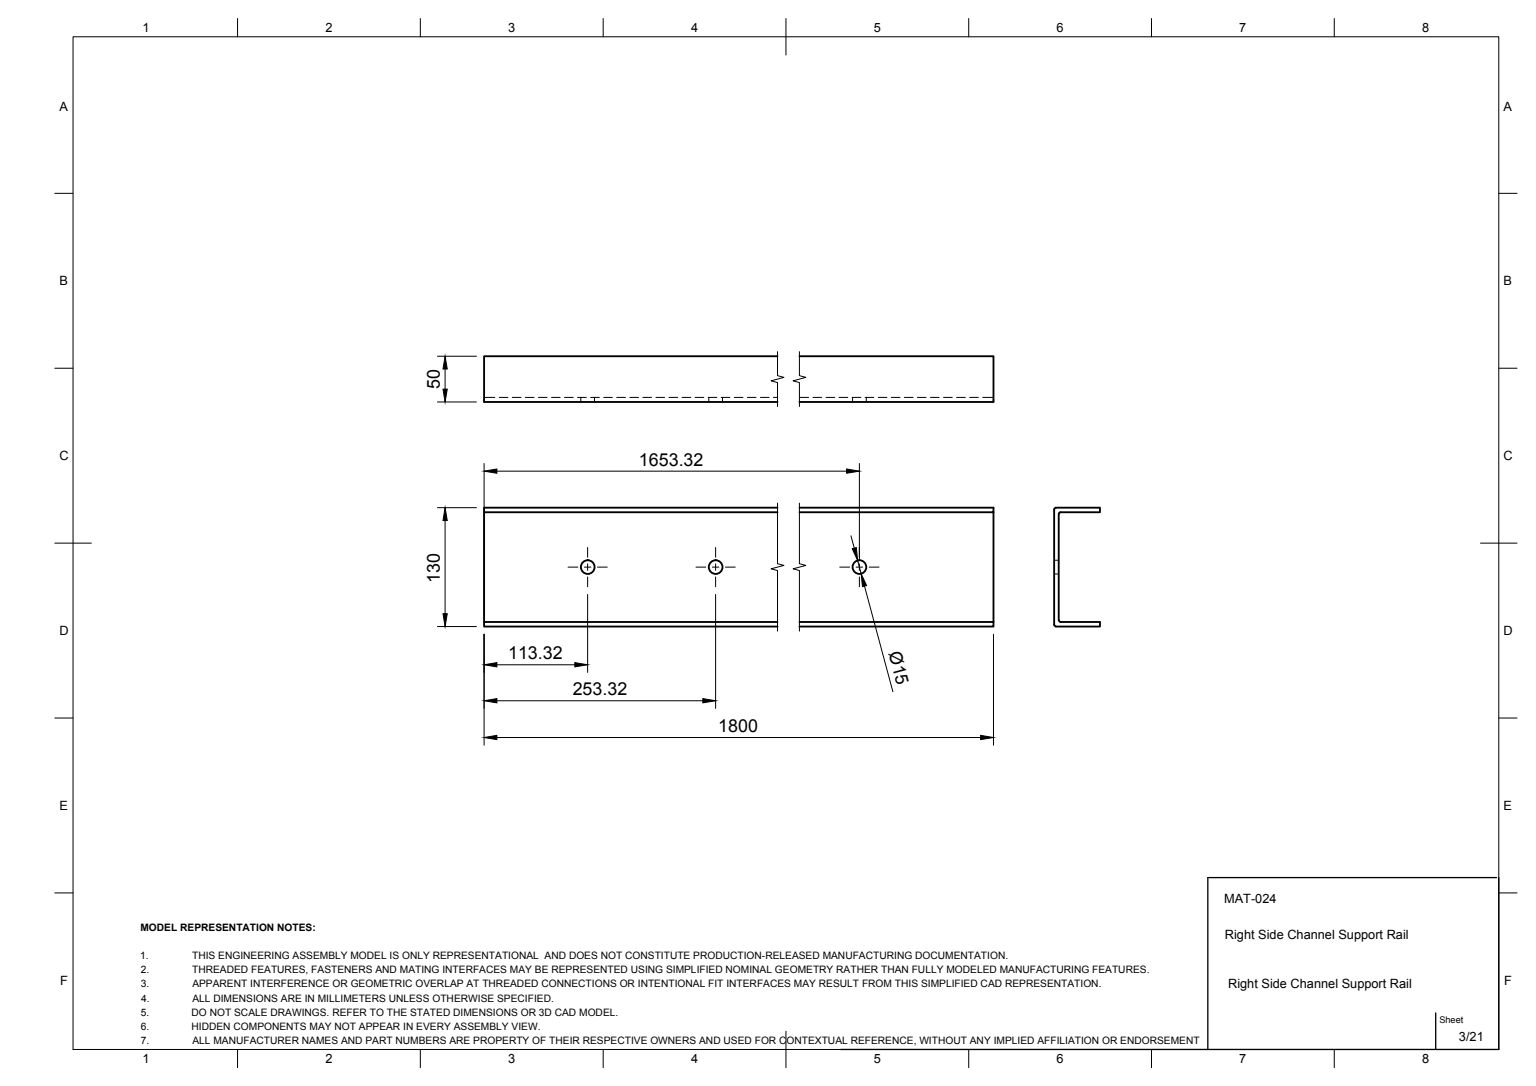
ISO-10303-21;
HEADER;
/* Generated by software containing ST-Developer
 * from STEP Tools, Inc. (www.steptools.com) 
 */

FILE_DESCRIPTION(
/* description */ ('STEP AP214'),
/* implementation_level */ '2;1');

FILE_NAME(
/* name */ 'Right Side Channel Support Rail.step',
/* time_stamp */ '2026-11-14T06:34:07-08:00',
/* author */ (''),
/* organization */ (''),
/* preprocessor_version */ 'ST-DEVELOPER v20.2',
/* originating_system */ 'Autodesk Translation Framework v15.17.0.0',
/* authorisation */ '');

FILE_SCHEMA (('AUTOMOTIVE_DESIGN { 1 0 10303 214 3 1 1 }'));
ENDSEC;

DATA;
#10=MECHANICAL_DESIGN_GEOMETRIC_PRESENTATION_REPRESENTATION('',(#7256),#310623);
#7222=SHAPE_REPRESENTATION_RELATIONSHIP('SRR','None',#310894,#7239);
#7239=ADVANCED_BREP_SHAPE_REPRESENTATION('',(#7324),#310603);
#7256=STYLED_ITEM('',(#311003),#7324);
#7324=MANIFOLD_SOLID_BREP('Body1',#93706);
#7391=FACE_BOUND('',#14442,.T.);
#7392=FACE_BOUND('',#14443,.T.);
#7393=FACE_BOUND('',#14444,.T.);
#7394=FACE_BOUND('',#14445,.T.);
#7395=FACE_BOUND('',#14446,.T.);
#7396=FACE_BOUND('',#14447,.T.);
#7397=FACE_BOUND('',#14448,.T.);
#7398=FACE_BOUND('',#14449,.T.);
#7399=FACE_BOUND('',#14450,.T.);
#7400=FACE_BOUND('',#14451,.T.);
#7401=FACE_BOUND('',#14452,.T.);
#7402=FACE_BOUND('',#14453,.T.);
#7403=FACE_BOUND('',#14458,.T.);
#7404=FACE_BOUND('',#14459,.T.);
#7405=FACE_BOUND('',#14460,.T.);
#7406=FACE_BOUND('',#14461,.T.);
#7407=FACE_BOUND('',#14462,.T.);
#7408=FACE_BOUND('',#14463,.T.);
#7409=FACE_BOUND('',#14464,.T.);
#7410=FACE_BOUND('',#14465,.T.);
#7411=FACE_BOUND('',#14466,.T.);
#7412=FACE_BOUND('',#14467,.T.);
#7413=FACE_BOUND('',#14468,.T.);
#7414=FACE_BOUND('',#14469,.T.);
#7706=PLANE('',#94001);
#7707=PLANE('',#94002);
#7708=PLANE('',#94003);
#7709=PLANE('',#94004);
#7710=PLANE('',#94005);
#7711=PLANE('',#94006);
#7712=PLANE('',#94007);
#7713=PLANE('',#94008);
#7714=PLANE('',#94009);
#7715=PLANE('',#94014);
#8688=FACE_OUTER_BOUND('',#14427,.T.);
#8689=FACE_OUTER_BOUND('',#14428,.T.);
#8690=FACE_OUTER_BOUND('',#14429,.T.);
#8691=FACE_OUTER_BOUND('',#14430,.T.);
#8692=FACE_OUTER_BOUND('',#14431,.T.);
#8693=FACE_OUTER_BOUND('',#14432,.T.);
#8694=FACE_OUTER_BOUND('',#14433,.T.);
#8695=FACE_OUTER_BOUND('',#14434,.T.);
#8696=FACE_OUTER_BOUND('',#14435,.T.);
#8697=FACE_OUTER_BOUND('',#14436,.T.);
#8698=FACE_OUTER_BOUND('',#14437,.T.);
#8699=FACE_OUTER_BOUND('',#14438,.T.);
#8700=FACE_OUTER_BOUND('',#14439,.T.);
#8701=FACE_OUTER_BOUND('',#14440,.T.);
#8702=FACE_OUTER_BOUND('',#14441,.T.);
#8703=FACE_OUTER_BOUND('',#14454,.T.);
#8704=FACE_OUTER_BOUND('',#14455,.T.);
#8705=FACE_OUTER_BOUND('',#14456,.T.);
#8706=FACE_OUTER_BOUND('',#14457,.T.);
#8707=FACE_OUTER_BOUND('',#14470,.T.);
#8708=FACE_OUTER_BOUND('',#14471,.T.);
#8709=FACE_OUTER_BOUND('',#14472,.T.);
#8710=FACE_OUTER_BOUND('',#14473,.T.);
#8711=FACE_OUTER_BOUND('',#14474,.T.);
#8712=FACE_OUTER_BOUND('',#14475,.T.);
#8713=FACE_OUTER_BOUND('',#14476,.T.);
#14427=EDGE_LOOP('',(#57657,#57658,#57659,#57660));
#14428=EDGE_LOOP('',(#57661,#57662,#57663,#57664));
#14429=EDGE_LOOP('',(#57665,#57666,#57667,#57668));
#14430=EDGE_LOOP('',(#57669,#57670,#57671,#57672));
#14431=EDGE_LOOP('',(#57673,#57674,#57675,#57676));
#14432=EDGE_LOOP('',(#57677,#57678,#57679,#57680));
#14433=EDGE_LOOP('',(#57681,#57682,#57683,#57684));
#14434=EDGE_LOOP('',(#57685,#57686,#57687,#57688));
#14435=EDGE_LOOP('',(#57689,#57690,#57691,#57692));
#14436=EDGE_LOOP('',(#57693,#57694,#57695,#57696));
#14437=EDGE_LOOP('',(#57697,#57698,#57699,#57700));
#14438=EDGE_LOOP('',(#57701,#57702,#57703,#57704));
#14439=EDGE_LOOP('',(#57705,#57706,#57707,#57708));
#14440=EDGE_LOOP('',(#57709,#57710,#57711,#57712));
#14441=EDGE_LOOP('',(#57713,#57714,#57715,#57716));
#14442=EDGE_LOOP('',(#57717));
#14443=EDGE_LOOP('',(#57718));
#14444=EDGE_LOOP('',(#57719));
#14445=EDGE_LOOP('',(#57720));
#14446=EDGE_LOOP('',(#57721));
#14447=EDGE_LOOP('',(#57722));
#14448=EDGE_LOOP('',(#57723));
#14449=EDGE_LOOP('',(#57724));
#14450=EDGE_LOOP('',(#57725));
#14451=EDGE_LOOP('',(#57726));
#14452=EDGE_LOOP('',(#57727));
#14453=EDGE_LOOP('',(#57728));
#14454=EDGE_LOOP('',(#57729,#57730,#57731,#57732));
#14455=EDGE_LOOP('',(#57733,#57734,#57735,#57736));
#14456=EDGE_LOOP('',(#57737,#57738,#57739,#57740));
#14457=EDGE_LOOP('',(#57741,#57742,#57743,#57744));
#14458=EDGE_LOOP('',(#57745));
#14459=EDGE_LOOP('',(#57746));
#14460=EDGE_LOOP('',(#57747));
#14461=EDGE_LOOP('',(#57748));
#14462=EDGE_LOOP('',(#57749));
#14463=EDGE_LOOP('',(#57750));
#14464=EDGE_LOOP('',(#57751));
#14465=EDGE_LOOP('',(#57752));
#14466=EDGE_LOOP('',(#57753));
#14467=EDGE_LOOP('',(#57754));
#14468=EDGE_LOOP('',(#57755));
#14469=EDGE_LOOP('',(#57756));
#14470=EDGE_LOOP('',(#57757,#57758,#57759,#57760));
#14471=EDGE_LOOP('',(#57761,#57762,#57763,#57764,#57765,#57766,#57767,#57768,
#57769,#57770,#57771,#57772));
#14472=EDGE_LOOP('',(#57773,#57774,#57775,#57776,#57777,#57778,#57779,#57780,
#57781,#57782,#57783,#57784));
#14473=EDGE_LOOP('',(#57785,#57786,#57787,#57788));
#14474=EDGE_LOOP('',(#57789,#57790,#57791,#57792));
#14475=EDGE_LOOP('',(#57793,#57794,#57795,#57796));
#14476=EDGE_LOOP('',(#57797,#57798,#57799,#57800));
#20481=LINE('',#131019,#24828);
#20482=LINE('',#131025,#24829);
#20483=LINE('',#131031,#24830);
#20484=LINE('',#131037,#24831);
#20485=LINE('',#131043,#24832);
#20486=LINE('',#131049,#24833);
#20487=LINE('',#131055,#24834);
#20488=LINE('',#131061,#24835);
#20489=LINE('',#131067,#24836);
#20490=LINE('',#131073,#24837);
#20491=LINE('',#131079,#24838);
#20492=LINE('',#131085,#24839);
#20493=LINE('',#131090,#24840);
#20494=LINE('',#131092,#24841);
#20495=LINE('',#131094,#24842);
#20496=LINE('',#131095,#24843);
#20497=LINE('',#131098,#24844);
#20498=LINE('',#131100,#24845);
#20499=LINE('',#131101,#24846);
#20500=LINE('',#131105,#24847);
#20501=LINE('',#131107,#24848);
#20502=LINE('',#131109,#24849);
#20503=LINE('',#131110,#24850);
#20504=LINE('',#131114,#24851);
#20505=LINE('',#131116,#24852);
#20506=LINE('',#131118,#24853);
#20507=LINE('',#131119,#24854);
#20508=LINE('',#131122,#24855);
#20509=LINE('',#131124,#24856);
#20510=LINE('',#131125,#24857);
#20511=LINE('',#131128,#24858);
#20512=LINE('',#131130,#24859);
#20513=LINE('',#131131,#24860);
#20514=LINE('',#131135,#24861);
#20515=LINE('',#131137,#24862);
#20516=LINE('',#131139,#24863);
#20517=LINE('',#131140,#24864);
#20518=LINE('',#131143,#24865);
#20519=LINE('',#131145,#24866);
#20520=LINE('',#131146,#24867);
#24828=VECTOR('',#104872,7.5);
#24829=VECTOR('',#104879,7.5);
#24830=VECTOR('',#104886,7.50000000000001);
#24831=VECTOR('',#104893,7.5);
#24832=VECTOR('',#104900,7.50000000000001);
#24833=VECTOR('',#104907,7.5);
#24834=VECTOR('',#104914,7.5);
#24835=VECTOR('',#104921,7.5);
#24836=VECTOR('',#104928,7.5);
#24837=VECTOR('',#104935,7.5);
#24838=VECTOR('',#104942,7.5);
#24839=VECTOR('',#104949,7.50000000000001);
#24840=VECTOR('',#104954,1000.);
#24841=VECTOR('',#104955,1000.);
#24842=VECTOR('',#104956,1000.);
#24843=VECTOR('',#104957,1000.);
#24844=VECTOR('',#104960,1000.);
#24845=VECTOR('',#104961,1000.);
#24846=VECTOR('',#104962,1000.);
#24847=VECTOR('',#104965,1000.);
#24848=VECTOR('',#104966,1000.);
#24849=VECTOR('',#104967,1000.);
#24850=VECTOR('',#104968,1000.);
#24851=VECTOR('',#104971,1000.);
#24852=VECTOR('',#104972,1000.);
#24853=VECTOR('',#104973,1000.);
#24854=VECTOR('',#104974,1000.);
#24855=VECTOR('',#104977,1000.);
#24856=VECTOR('',#104978,1000.);
#24857=VECTOR('',#104979,1000.);
#24858=VECTOR('',#104982,1000.);
#24859=VECTOR('',#104983,1000.);
#24860=VECTOR('',#104984,1000.);
#24861=VECTOR('',#104987,1000.);
#24862=VECTOR('',#104988,1000.);
#24863=VECTOR('',#104989,1000.);
#24864=VECTOR('',#104990,1000.);
#24865=VECTOR('',#104993,1000.);
#24866=VECTOR('',#104994,1000.);
#24867=VECTOR('',#104995,1000.);
#29175=CIRCLE('',#93966,7.5);
#29176=CIRCLE('',#93967,7.5);
#29177=CIRCLE('',#93969,7.5);
#29178=CIRCLE('',#93970,7.5);
#29179=CIRCLE('',#93972,7.50000000000001);
#29180=CIRCLE('',#93973,7.50000000000001);
#29181=CIRCLE('',#93975,7.5);
#29182=CIRCLE('',#93976,7.5);
#29183=CIRCLE('',#93978,7.50000000000001);
#29184=CIRCLE('',#93979,7.50000000000001);
#29185=CIRCLE('',#93981,7.5);
#29186=CIRCLE('',#93982,7.5);
#29187=CIRCLE('',#93984,7.5);
#29188=CIRCLE('',#93985,7.5);
#29189=CIRCLE('',#93987,7.5);
#29190=CIRCLE('',#93988,7.5);
#29191=CIRCLE('',#93990,7.5);
#29192=CIRCLE('',#93991,7.5);
#29193=CIRCLE('',#93993,7.5);
#29194=CIRCLE('',#93994,7.5);
#29195=CIRCLE('',#93996,7.5);
#29196=CIRCLE('',#93997,7.5);
#29197=CIRCLE('',#93999,7.50000000000001);
#29198=CIRCLE('',#94000,7.50000000000001);
#29199=CIRCLE('',#94010,2.);
#29200=CIRCLE('',#94011,2.);
#29201=CIRCLE('',#94012,2.);
#29202=CIRCLE('',#94013,2.);
#29203=CIRCLE('',#94015,2.);
#29204=CIRCLE('',#94016,2.);
#29205=CIRCLE('',#94017,2.);
#29206=CIRCLE('',#94018,2.);
#35105=VERTEX_POINT('',#131016);
#35106=VERTEX_POINT('',#131018);
#35107=VERTEX_POINT('',#131022);
#35108=VERTEX_POINT('',#131024);
#35109=VERTEX_POINT('',#131028);
#35110=VERTEX_POINT('',#131030);
#35111=VERTEX_POINT('',#131034);
#35112=VERTEX_POINT('',#131036);
#35113=VERTEX_POINT('',#131040);
#35114=VERTEX_POINT('',#131042);
#35115=VERTEX_POINT('',#131046);
#35116=VERTEX_POINT('',#131048);
#35117=VERTEX_POINT('',#131052);
#35118=VERTEX_POINT('',#131054);
#35119=VERTEX_POINT('',#131058);
#35120=VERTEX_POINT('',#131060);
#35121=VERTEX_POINT('',#131064);
#35122=VERTEX_POINT('',#131066);
#35123=VERTEX_POINT('',#131070);
#35124=VERTEX_POINT('',#131072);
#35125=VERTEX_POINT('',#131076);
#35126=VERTEX_POINT('',#131078);
#35127=VERTEX_POINT('',#131082);
#35128=VERTEX_POINT('',#131084);
#35129=VERTEX_POINT('',#131088);
#35130=VERTEX_POINT('',#131089);
#35131=VERTEX_POINT('',#131091);
#35132=VERTEX_POINT('',#131093);
#35133=VERTEX_POINT('',#131097);
#35134=VERTEX_POINT('',#131099);
#35135=VERTEX_POINT('',#131103);
#35136=VERTEX_POINT('',#131104);
#35137=VERTEX_POINT('',#131106);
#35138=VERTEX_POINT('',#131108);
#35139=VERTEX_POINT('',#131112);
#35140=VERTEX_POINT('',#131113);
#35141=VERTEX_POINT('',#131115);
#35142=VERTEX_POINT('',#131117);
#35143=VERTEX_POINT('',#131121);
#35144=VERTEX_POINT('',#131123);
#35145=VERTEX_POINT('',#131127);
#35146=VERTEX_POINT('',#131129);
#35147=VERTEX_POINT('',#131133);
#35148=VERTEX_POINT('',#131134);
#35149=VERTEX_POINT('',#131136);
#35150=VERTEX_POINT('',#131138);
#35151=VERTEX_POINT('',#131142);
#35152=VERTEX_POINT('',#131144);
#43608=EDGE_CURVE('',#35105,#35105,#29175,.T.);
#43609=EDGE_CURVE('',#35105,#35106,#20481,.T.);
#43610=EDGE_CURVE('',#35106,#35106,#29176,.T.);
#43611=EDGE_CURVE('',#35107,#35107,#29177,.T.);
#43612=EDGE_CURVE('',#35107,#35108,#20482,.T.);
#43613=EDGE_CURVE('',#35108,#35108,#29178,.T.);
#43614=EDGE_CURVE('',#35109,#35109,#29179,.T.);
#43615=EDGE_CURVE('',#35109,#35110,#20483,.T.);
#43616=EDGE_CURVE('',#35110,#35110,#29180,.T.);
#43617=EDGE_CURVE('',#35111,#35111,#29181,.T.);
#43618=EDGE_CURVE('',#35111,#35112,#20484,.T.);
#43619=EDGE_CURVE('',#35112,#35112,#29182,.T.);
#43620=EDGE_CURVE('',#35113,#35113,#29183,.T.);
#43621=EDGE_CURVE('',#35113,#35114,#20485,.T.);
#43622=EDGE_CURVE('',#35114,#35114,#29184,.T.);
#43623=EDGE_CURVE('',#35115,#35115,#29185,.T.);
#43624=EDGE_CURVE('',#35115,#35116,#20486,.T.);
#43625=EDGE_CURVE('',#35116,#35116,#29186,.T.);
#43626=EDGE_CURVE('',#35117,#35117,#29187,.T.);
#43627=EDGE_CURVE('',#35117,#35118,#20487,.T.);
#43628=EDGE_CURVE('',#35118,#35118,#29188,.T.);
#43629=EDGE_CURVE('',#35119,#35119,#29189,.T.);
#43630=EDGE_CURVE('',#35119,#35120,#20488,.T.);
#43631=EDGE_CURVE('',#35120,#35120,#29190,.T.);
#43632=EDGE_CURVE('',#35121,#35121,#29191,.T.);
#43633=EDGE_CURVE('',#35121,#35122,#20489,.T.);
#43634=EDGE_CURVE('',#35122,#35122,#29192,.T.);
#43635=EDGE_CURVE('',#35123,#35123,#29193,.T.);
#43636=EDGE_CURVE('',#35123,#35124,#20490,.T.);
#43637=EDGE_CURVE('',#35124,#35124,#29194,.T.);
#43638=EDGE_CURVE('',#35125,#35125,#29195,.T.);
#43639=EDGE_CURVE('',#35125,#35126,#20491,.T.);
#43640=EDGE_CURVE('',#35126,#35126,#29196,.T.);
#43641=EDGE_CURVE('',#35127,#35127,#29197,.T.);
#43642=EDGE_CURVE('',#35127,#35128,#20492,.T.);
#43643=EDGE_CURVE('',#35128,#35128,#29198,.T.);
#43644=EDGE_CURVE('',#35129,#35130,#20493,.T.);
#43645=EDGE_CURVE('',#35131,#35130,#20494,.T.);
#43646=EDGE_CURVE('',#35132,#35131,#20495,.T.);
#43647=EDGE_CURVE('',#35132,#35129,#20496,.T.);
#43648=EDGE_CURVE('',#35130,#35133,#20497,.T.);
#43649=EDGE_CURVE('',#35133,#35134,#20498,.T.);
#43650=EDGE_CURVE('',#35131,#35134,#20499,.T.);
#43651=EDGE_CURVE('',#35135,#35136,#20500,.T.);
#43652=EDGE_CURVE('',#35136,#35137,#20501,.T.);
#43653=EDGE_CURVE('',#35138,#35137,#20502,.T.);
#43654=EDGE_CURVE('',#35138,#35135,#20503,.T.);
#43655=EDGE_CURVE('',#35139,#35140,#20504,.T.);
#43656=EDGE_CURVE('',#35139,#35141,#20505,.T.);
#43657=EDGE_CURVE('',#35141,#35142,#20506,.T.);
#43658=EDGE_CURVE('',#35140,#35142,#20507,.T.);
#43659=EDGE_CURVE('',#35142,#35143,#20508,.T.);
#43660=EDGE_CURVE('',#35144,#35143,#20509,.T.);
#43661=EDGE_CURVE('',#35140,#35144,#20510,.T.);
#43662=EDGE_CURVE('',#35143,#35145,#20511,.T.);
#43663=EDGE_CURVE('',#35145,#35146,#20512,.T.);
#43664=EDGE_CURVE('',#35144,#35146,#20513,.T.);
#43665=EDGE_CURVE('',#35147,#35148,#20514,.T.);
#43666=EDGE_CURVE('',#35148,#35149,#20515,.T.);
#43667=EDGE_CURVE('',#35150,#35149,#20516,.T.);
#43668=EDGE_CURVE('',#35150,#35147,#20517,.T.);
#43669=EDGE_CURVE('',#35151,#35132,#20518,.T.);
#43670=EDGE_CURVE('',#35151,#35152,#20519,.T.);
#43671=EDGE_CURVE('',#35152,#35129,#20520,.T.);
#43672=EDGE_CURVE('',#35137,#35139,#29199,.T.);
#43673=EDGE_CURVE('',#35146,#35150,#29200,.T.);
#43674=EDGE_CURVE('',#35149,#35151,#29201,.T.);
#43675=EDGE_CURVE('',#35134,#35138,#29202,.T.);
#43676=EDGE_CURVE('',#35141,#35136,#29203,.T.);
#43677=EDGE_CURVE('',#35135,#35133,#29204,.T.);
#43678=EDGE_CURVE('',#35152,#35148,#29205,.T.);
#43679=EDGE_CURVE('',#35147,#35145,#29206,.T.);
#57657=ORIENTED_EDGE('',*,*,#43608,.F.);
#57658=ORIENTED_EDGE('',*,*,#43609,.T.);
#57659=ORIENTED_EDGE('',*,*,#43610,.T.);
#57660=ORIENTED_EDGE('',*,*,#43609,.F.);
#57661=ORIENTED_EDGE('',*,*,#43611,.F.);
#57662=ORIENTED_EDGE('',*,*,#43612,.T.);
#57663=ORIENTED_EDGE('',*,*,#43613,.T.);
#57664=ORIENTED_EDGE('',*,*,#43612,.F.);
#57665=ORIENTED_EDGE('',*,*,#43614,.F.);
#57666=ORIENTED_EDGE('',*,*,#43615,.T.);
#57667=ORIENTED_EDGE('',*,*,#43616,.T.);
#57668=ORIENTED_EDGE('',*,*,#43615,.F.);
#57669=ORIENTED_EDGE('',*,*,#43617,.F.);
#57670=ORIENTED_EDGE('',*,*,#43618,.T.);
#57671=ORIENTED_EDGE('',*,*,#43619,.T.);
#57672=ORIENTED_EDGE('',*,*,#43618,.F.);
#57673=ORIENTED_EDGE('',*,*,#43620,.F.);
#57674=ORIENTED_EDGE('',*,*,#43621,.T.);
#57675=ORIENTED_EDGE('',*,*,#43622,.T.);
#57676=ORIENTED_EDGE('',*,*,#43621,.F.);
#57677=ORIENTED_EDGE('',*,*,#43623,.F.);
#57678=ORIENTED_EDGE('',*,*,#43624,.T.);
#57679=ORIENTED_EDGE('',*,*,#43625,.T.);
#57680=ORIENTED_EDGE('',*,*,#43624,.F.);
#57681=ORIENTED_EDGE('',*,*,#43626,.F.);
#57682=ORIENTED_EDGE('',*,*,#43627,.T.);
#57683=ORIENTED_EDGE('',*,*,#43628,.T.);
#57684=ORIENTED_EDGE('',*,*,#43627,.F.);
#57685=ORIENTED_EDGE('',*,*,#43629,.F.);
#57686=ORIENTED_EDGE('',*,*,#43630,.T.);
#57687=ORIENTED_EDGE('',*,*,#43631,.T.);
#57688=ORIENTED_EDGE('',*,*,#43630,.F.);
#57689=ORIENTED_EDGE('',*,*,#43632,.F.);
#57690=ORIENTED_EDGE('',*,*,#43633,.T.);
#57691=ORIENTED_EDGE('',*,*,#43634,.T.);
#57692=ORIENTED_EDGE('',*,*,#43633,.F.);
#57693=ORIENTED_EDGE('',*,*,#43635,.F.);
#57694=ORIENTED_EDGE('',*,*,#43636,.T.);
#57695=ORIENTED_EDGE('',*,*,#43637,.T.);
#57696=ORIENTED_EDGE('',*,*,#43636,.F.);
#57697=ORIENTED_EDGE('',*,*,#43638,.F.);
#57698=ORIENTED_EDGE('',*,*,#43639,.T.);
#57699=ORIENTED_EDGE('',*,*,#43640,.T.);
#57700=ORIENTED_EDGE('',*,*,#43639,.F.);
#57701=ORIENTED_EDGE('',*,*,#43641,.F.);
#57702=ORIENTED_EDGE('',*,*,#43642,.T.);
#57703=ORIENTED_EDGE('',*,*,#43643,.T.);
#57704=ORIENTED_EDGE('',*,*,#43642,.F.);
#57705=ORIENTED_EDGE('',*,*,#43644,.T.);
#57706=ORIENTED_EDGE('',*,*,#43645,.F.);
#57707=ORIENTED_EDGE('',*,*,#43646,.F.);
#57708=ORIENTED_EDGE('',*,*,#43647,.T.);
#57709=ORIENTED_EDGE('',*,*,#43648,.T.);
#57710=ORIENTED_EDGE('',*,*,#43649,.T.);
#57711=ORIENTED_EDGE('',*,*,#43650,.F.);
#57712=ORIENTED_EDGE('',*,*,#43645,.T.);
#57713=ORIENTED_EDGE('',*,*,#43651,.T.);
#57714=ORIENTED_EDGE('',*,*,#43652,.T.);
#57715=ORIENTED_EDGE('',*,*,#43653,.F.);
#57716=ORIENTED_EDGE('',*,*,#43654,.T.);
#57717=ORIENTED_EDGE('',*,*,#43608,.T.);
#57718=ORIENTED_EDGE('',*,*,#43611,.T.);
#57719=ORIENTED_EDGE('',*,*,#43614,.T.);
#57720=ORIENTED_EDGE('',*,*,#43617,.T.);
#57721=ORIENTED_EDGE('',*,*,#43620,.T.);
#57722=ORIENTED_EDGE('',*,*,#43623,.T.);
#57723=ORIENTED_EDGE('',*,*,#43626,.T.);
#57724=ORIENTED_EDGE('',*,*,#43629,.T.);
#57725=ORIENTED_EDGE('',*,*,#43632,.T.);
#57726=ORIENTED_EDGE('',*,*,#43635,.T.);
#57727=ORIENTED_EDGE('',*,*,#43638,.T.);
#57728=ORIENTED_EDGE('',*,*,#43641,.T.);
#57729=ORIENTED_EDGE('',*,*,#43655,.F.);
#57730=ORIENTED_EDGE('',*,*,#43656,.T.);
#57731=ORIENTED_EDGE('',*,*,#43657,.T.);
#57732=ORIENTED_EDGE('',*,*,#43658,.F.);
#57733=ORIENTED_EDGE('',*,*,#43659,.T.);
#57734=ORIENTED_EDGE('',*,*,#43660,.F.);
#57735=ORIENTED_EDGE('',*,*,#43661,.F.);
#57736=ORIENTED_EDGE('',*,*,#43658,.T.);
#57737=ORIENTED_EDGE('',*,*,#43662,.T.);
#57738=ORIENTED_EDGE('',*,*,#43663,.T.);
#57739=ORIENTED_EDGE('',*,*,#43664,.F.);
#57740=ORIENTED_EDGE('',*,*,#43660,.T.);
#57741=ORIENTED_EDGE('',*,*,#43665,.T.);
#57742=ORIENTED_EDGE('',*,*,#43666,.T.);
#57743=ORIENTED_EDGE('',*,*,#43667,.F.);
#57744=ORIENTED_EDGE('',*,*,#43668,.T.);
#57745=ORIENTED_EDGE('',*,*,#43610,.F.);
#57746=ORIENTED_EDGE('',*,*,#43613,.F.);
#57747=ORIENTED_EDGE('',*,*,#43616,.F.);
#57748=ORIENTED_EDGE('',*,*,#43619,.F.);
#57749=ORIENTED_EDGE('',*,*,#43622,.F.);
#57750=ORIENTED_EDGE('',*,*,#43625,.F.);
#57751=ORIENTED_EDGE('',*,*,#43628,.F.);
#57752=ORIENTED_EDGE('',*,*,#43631,.F.);
#57753=ORIENTED_EDGE('',*,*,#43634,.F.);
#57754=ORIENTED_EDGE('',*,*,#43637,.F.);
#57755=ORIENTED_EDGE('',*,*,#43640,.F.);
#57756=ORIENTED_EDGE('',*,*,#43643,.F.);
#57757=ORIENTED_EDGE('',*,*,#43669,.F.);
#57758=ORIENTED_EDGE('',*,*,#43670,.T.);
#57759=ORIENTED_EDGE('',*,*,#43671,.T.);
#57760=ORIENTED_EDGE('',*,*,#43647,.F.);
#57761=ORIENTED_EDGE('',*,*,#43653,.T.);
#57762=ORIENTED_EDGE('',*,*,#43672,.T.);
#57763=ORIENTED_EDGE('',*,*,#43655,.T.);
#57764=ORIENTED_EDGE('',*,*,#43661,.T.);
#57765=ORIENTED_EDGE('',*,*,#43664,.T.);
#57766=ORIENTED_EDGE('',*,*,#43673,.T.);
#57767=ORIENTED_EDGE('',*,*,#43667,.T.);
#57768=ORIENTED_EDGE('',*,*,#43674,.T.);
#57769=ORIENTED_EDGE('',*,*,#43669,.T.);
#57770=ORIENTED_EDGE('',*,*,#43646,.T.);
#57771=ORIENTED_EDGE('',*,*,#43650,.T.);
#57772=ORIENTED_EDGE('',*,*,#43675,.T.);
#57773=ORIENTED_EDGE('',*,*,#43657,.F.);
#57774=ORIENTED_EDGE('',*,*,#43676,.T.);
#57775=ORIENTED_EDGE('',*,*,#43651,.F.);
#57776=ORIENTED_EDGE('',*,*,#43677,.T.);
#57777=ORIENTED_EDGE('',*,*,#43648,.F.);
#57778=ORIENTED_EDGE('',*,*,#43644,.F.);
#57779=ORIENTED_EDGE('',*,*,#43671,.F.);
#57780=ORIENTED_EDGE('',*,*,#43678,.T.);
#57781=ORIENTED_EDGE('',*,*,#43665,.F.);
#57782=ORIENTED_EDGE('',*,*,#43679,.T.);
#57783=ORIENTED_EDGE('',*,*,#43662,.F.);
#57784=ORIENTED_EDGE('',*,*,#43659,.F.);
#57785=ORIENTED_EDGE('',*,*,#43672,.F.);
#57786=ORIENTED_EDGE('',*,*,#43652,.F.);
#57787=ORIENTED_EDGE('',*,*,#43676,.F.);
#57788=ORIENTED_EDGE('',*,*,#43656,.F.);
#57789=ORIENTED_EDGE('',*,*,#43675,.F.);
#57790=ORIENTED_EDGE('',*,*,#43649,.F.);
#57791=ORIENTED_EDGE('',*,*,#43677,.F.);
#57792=ORIENTED_EDGE('',*,*,#43654,.F.);
#57793=ORIENTED_EDGE('',*,*,#43674,.F.);
#57794=ORIENTED_EDGE('',*,*,#43666,.F.);
#57795=ORIENTED_EDGE('',*,*,#43678,.F.);
#57796=ORIENTED_EDGE('',*,*,#43670,.F.);
#57797=ORIENTED_EDGE('',*,*,#43673,.F.);
#57798=ORIENTED_EDGE('',*,*,#43663,.F.);
#57799=ORIENTED_EDGE('',*,*,#43679,.F.);
#57800=ORIENTED_EDGE('',*,*,#43668,.F.);
#85755=CYLINDRICAL_SURFACE('',#93965,7.5);
#85756=CYLINDRICAL_SURFACE('',#93968,7.5);
#85757=CYLINDRICAL_SURFACE('',#93971,7.50000000000001);
#85758=CYLINDRICAL_SURFACE('',#93974,7.5);
#85759=CYLINDRICAL_SURFACE('',#93977,7.50000000000001);
#85760=CYLINDRICAL_SURFACE('',#93980,7.5);
#85761=CYLINDRICAL_SURFACE('',#93983,7.5);
#85762=CYLINDRICAL_SURFACE('',#93986,7.5);
#85763=CYLINDRICAL_SURFACE('',#93989,7.5);
#85764=CYLINDRICAL_SURFACE('',#93992,7.5);
#85765=CYLINDRICAL_SURFACE('',#93995,7.5);
#85766=CYLINDRICAL_SURFACE('',#93998,7.50000000000001);
#85767=CYLINDRICAL_SURFACE('',#94019,2.);
#85768=CYLINDRICAL_SURFACE('',#94020,2.);
#85769=CYLINDRICAL_SURFACE('',#94021,2.);
#85770=CYLINDRICAL_SURFACE('',#94022,2.);
#87967=ADVANCED_FACE('',(#8688),#85755,.F.);
#87968=ADVANCED_FACE('',(#8689),#85756,.F.);
#87969=ADVANCED_FACE('',(#8690),#85757,.F.);
#87970=ADVANCED_FACE('',(#8691),#85758,.F.);
#87971=ADVANCED_FACE('',(#8692),#85759,.F.);
#87972=ADVANCED_FACE('',(#8693),#85760,.F.);
#87973=ADVANCED_FACE('',(#8694),#85761,.F.);
#87974=ADVANCED_FACE('',(#8695),#85762,.F.);
#87975=ADVANCED_FACE('',(#8696),#85763,.F.);
#87976=ADVANCED_FACE('',(#8697),#85764,.F.);
#87977=ADVANCED_FACE('',(#8698),#85765,.F.);
#87978=ADVANCED_FACE('',(#8699),#85766,.F.);
#87979=ADVANCED_FACE('',(#8700),#7706,.F.);
#87980=ADVANCED_FACE('',(#8701),#7707,.F.);
#87981=ADVANCED_FACE('',(#8702,#7391,#7392,#7393,#7394,#7395,#7396,#7397,
#7398,#7399,#7400,#7401,#7402),#7708,.F.);
#87982=ADVANCED_FACE('',(#8703),#7709,.F.);
#87983=ADVANCED_FACE('',(#8704),#7710,.F.);
#87984=ADVANCED_FACE('',(#8705),#7711,.F.);
#87985=ADVANCED_FACE('',(#8706,#7403,#7404,#7405,#7406,#7407,#7408,#7409,
#7410,#7411,#7412,#7413,#7414),#7712,.F.);
#87986=ADVANCED_FACE('',(#8707),#7713,.F.);
#87987=ADVANCED_FACE('',(#8708),#7714,.T.);
#87988=ADVANCED_FACE('',(#8709),#7715,.F.);
#87989=ADVANCED_FACE('',(#8710),#85767,.T.);
#87990=ADVANCED_FACE('',(#8711),#85768,.T.);
#87991=ADVANCED_FACE('',(#8712),#85769,.F.);
#87992=ADVANCED_FACE('',(#8713),#85770,.F.);
#93706=CLOSED_SHELL('',(#87967,#87968,#87969,#87970,#87971,#87972,#87973,
#87974,#87975,#87976,#87977,#87978,#87979,#87980,#87981,#87982,#87983,#87984,
#87985,#87986,#87987,#87988,#87989,#87990,#87991,#87992));
#93964=AXIS2_PLACEMENT_3D('',#131014,#104866,#104867);
#93965=AXIS2_PLACEMENT_3D('',#131015,#104868,#104869);
#93966=AXIS2_PLACEMENT_3D('',#131017,#104870,#104871);
#93967=AXIS2_PLACEMENT_3D('',#131020,#104873,#104874);
#93968=AXIS2_PLACEMENT_3D('',#131021,#104875,#104876);
#93969=AXIS2_PLACEMENT_3D('',#131023,#104877,#104878);
#93970=AXIS2_PLACEMENT_3D('',#131026,#104880,#104881);
#93971=AXIS2_PLACEMENT_3D('',#131027,#104882,#104883);
#93972=AXIS2_PLACEMENT_3D('',#131029,#104884,#104885);
#93973=AXIS2_PLACEMENT_3D('',#131032,#104887,#104888);
#93974=AXIS2_PLACEMENT_3D('',#131033,#104889,#104890);
#93975=AXIS2_PLACEMENT_3D('',#131035,#104891,#104892);
#93976=AXIS2_PLACEMENT_3D('',#131038,#104894,#104895);
#93977=AXIS2_PLACEMENT_3D('',#131039,#104896,#104897);
#93978=AXIS2_PLACEMENT_3D('',#131041,#104898,#104899);
#93979=AXIS2_PLACEMENT_3D('',#131044,#104901,#104902);
#93980=AXIS2_PLACEMENT_3D('',#131045,#104903,#104904);
#93981=AXIS2_PLACEMENT_3D('',#131047,#104905,#104906);
#93982=AXIS2_PLACEMENT_3D('',#131050,#104908,#104909);
#93983=AXIS2_PLACEMENT_3D('',#131051,#104910,#104911);
#93984=AXIS2_PLACEMENT_3D('',#131053,#104912,#104913);
#93985=AXIS2_PLACEMENT_3D('',#131056,#104915,#104916);
#93986=AXIS2_PLACEMENT_3D('',#131057,#104917,#104918);
#93987=AXIS2_PLACEMENT_3D('',#131059,#104919,#104920);
#93988=AXIS2_PLACEMENT_3D('',#131062,#104922,#104923);
#93989=AXIS2_PLACEMENT_3D('',#131063,#104924,#104925);
#93990=AXIS2_PLACEMENT_3D('',#131065,#104926,#104927);
#93991=AXIS2_PLACEMENT_3D('',#131068,#104929,#104930);
#93992=AXIS2_PLACEMENT_3D('',#131069,#104931,#104932);
#93993=AXIS2_PLACEMENT_3D('',#131071,#104933,#104934);
#93994=AXIS2_PLACEMENT_3D('',#131074,#104936,#104937);
#93995=AXIS2_PLACEMENT_3D('',#131075,#104938,#104939);
#93996=AXIS2_PLACEMENT_3D('',#131077,#104940,#104941);
#93997=AXIS2_PLACEMENT_3D('',#131080,#104943,#104944);
#93998=AXIS2_PLACEMENT_3D('',#131081,#104945,#104946);
#93999=AXIS2_PLACEMENT_3D('',#131083,#104947,#104948);
#94000=AXIS2_PLACEMENT_3D('',#131086,#104950,#104951);
#94001=AXIS2_PLACEMENT_3D('',#131087,#104952,#104953);
#94002=AXIS2_PLACEMENT_3D('',#131096,#104958,#104959);
#94003=AXIS2_PLACEMENT_3D('',#131102,#104963,#104964);
#94004=AXIS2_PLACEMENT_3D('',#131111,#104969,#104970);
#94005=AXIS2_PLACEMENT_3D('',#131120,#104975,#104976);
#94006=AXIS2_PLACEMENT_3D('',#131126,#104980,#104981);
#94007=AXIS2_PLACEMENT_3D('',#131132,#104985,#104986);
#94008=AXIS2_PLACEMENT_3D('',#131141,#104991,#104992);
#94009=AXIS2_PLACEMENT_3D('',#131147,#104996,#104997);
#94010=AXIS2_PLACEMENT_3D('',#131148,#104998,#104999);
#94011=AXIS2_PLACEMENT_3D('',#131149,#105000,#105001);
#94012=AXIS2_PLACEMENT_3D('',#131150,#105002,#105003);
#94013=AXIS2_PLACEMENT_3D('',#131151,#105004,#105005);
#94014=AXIS2_PLACEMENT_3D('',#131152,#105006,#105007);
#94015=AXIS2_PLACEMENT_3D('',#131153,#105008,#105009);
#94016=AXIS2_PLACEMENT_3D('',#131154,#105010,#105011);
#94017=AXIS2_PLACEMENT_3D('',#131155,#105012,#105013);
#94018=AXIS2_PLACEMENT_3D('',#131156,#105014,#105015);
#94019=AXIS2_PLACEMENT_3D('',#131157,#105016,#105017);
#94020=AXIS2_PLACEMENT_3D('',#131158,#105018,#105019);
#94021=AXIS2_PLACEMENT_3D('',#131159,#105020,#105021);
#94022=AXIS2_PLACEMENT_3D('',#131160,#105022,#105023);
#104866=DIRECTION('axis',(0.,0.,1.));
#104867=DIRECTION('refdir',(1.,0.,0.));
#104868=DIRECTION('center_axis',(1.,0.,-2.89120579329468E-17));
#104869=DIRECTION('ref_axis',(-2.89120579329468E-17,0.,-1.));
#104870=DIRECTION('center_axis',(1.,0.,-5.33761069531325E-17));
#104871=DIRECTION('ref_axis',(-5.33761069531325E-17,0.,-1.));
#104872=DIRECTION('',(1.,0.,-2.89120579329468E-17));
#104873=DIRECTION('center_axis',(1.,0.,-2.89120579329468E-17));
#104874=DIRECTION('ref_axis',(-2.89120579329468E-17,0.,-1.));
#104875=DIRECTION('center_axis',(1.,0.,-2.89120579329468E-17));
#104876=DIRECTION('ref_axis',(-2.89120579329468E-17,0.,-1.));
#104877=DIRECTION('center_axis',(1.,0.,-5.33761069531325E-17));
#104878=DIRECTION('ref_axis',(-5.33761069531325E-17,0.,-1.));
#104879=DIRECTION('',(1.,0.,-2.89120579329468E-17));
#104880=DIRECTION('center_axis',(1.,0.,-2.89120579329468E-17));
#104881=DIRECTION('ref_axis',(-2.89120579329468E-17,0.,-1.));
#104882=DIRECTION('center_axis',(1.,0.,-2.89120579329468E-17));
#104883=DIRECTION('ref_axis',(-2.89120579329468E-17,0.,-1.));
#104884=DIRECTION('center_axis',(1.,0.,-5.33761069531325E-17));
#104885=DIRECTION('ref_axis',(-5.33761069531325E-17,0.,-1.));
#104886=DIRECTION('',(1.,0.,-2.89120579329468E-17));
#104887=DIRECTION('center_axis',(1.,0.,-2.89120579329468E-17));
#104888=DIRECTION('ref_axis',(-2.89120579329468E-17,0.,-1.));
#104889=DIRECTION('center_axis',(1.,0.,-2.89120579329468E-17));
#104890=DIRECTION('ref_axis',(-2.89120579329468E-17,0.,-1.));
#104891=DIRECTION('center_axis',(1.,0.,-5.33761069531325E-17));
#104892=DIRECTION('ref_axis',(-5.33761069531325E-17,0.,-1.));
#104893=DIRECTION('',(1.,0.,-2.89120579329468E-17));
#104894=DIRECTION('center_axis',(1.,0.,-2.89120579329468E-17));
#104895=DIRECTION('ref_axis',(-2.89120579329468E-17,0.,-1.));
#104896=DIRECTION('center_axis',(1.,0.,-2.89120579329468E-17));
#104897=DIRECTION('ref_axis',(-2.89120579329468E-17,0.,-1.));
#104898=DIRECTION('center_axis',(1.,0.,-5.33761069531325E-17));
#104899=DIRECTION('ref_axis',(-5.33761069531325E-17,0.,-1.));
#104900=DIRECTION('',(1.,0.,-2.89120579329468E-17));
#104901=DIRECTION('center_axis',(1.,0.,-2.89120579329468E-17));
#104902=DIRECTION('ref_axis',(-2.89120579329468E-17,0.,-1.));
#104903=DIRECTION('center_axis',(1.,0.,-2.89120579329468E-17));
#104904=DIRECTION('ref_axis',(-2.89120579329468E-17,0.,-1.));
#104905=DIRECTION('center_axis',(1.,0.,-5.33761069531325E-17));
#104906=DIRECTION('ref_axis',(-5.33761069531325E-17,0.,-1.));
#104907=DIRECTION('',(1.,0.,-2.89120579329468E-17));
#104908=DIRECTION('center_axis',(1.,0.,-2.89120579329468E-17));
#104909=DIRECTION('ref_axis',(-2.89120579329468E-17,0.,-1.));
#104910=DIRECTION('center_axis',(1.,0.,-2.89120579329468E-17));
#104911=DIRECTION('ref_axis',(-2.89120579329468E-17,0.,-1.));
#104912=DIRECTION('center_axis',(1.,0.,-5.33761069531325E-17));
#104913=DIRECTION('ref_axis',(-5.33761069531325E-17,0.,-1.));
#104914=DIRECTION('',(1.,0.,-2.89120579329468E-17));
#104915=DIRECTION('center_axis',(1.,0.,-2.89120579329468E-17));
#104916=DIRECTION('ref_axis',(-2.89120579329468E-17,0.,-1.));
#104917=DIRECTION('center_axis',(1.,0.,-2.89120579329468E-17));
#104918=DIRECTION('ref_axis',(-2.89120579329468E-17,0.,-1.));
#104919=DIRECTION('center_axis',(1.,0.,-5.33761069531325E-17));
#104920=DIRECTION('ref_axis',(-5.33761069531325E-17,0.,-1.));
#104921=DIRECTION('',(1.,0.,-2.89120579329468E-17));
#104922=DIRECTION('center_axis',(1.,0.,-2.89120579329468E-17));
#104923=DIRECTION('ref_axis',(-2.89120579329468E-17,0.,-1.));
#104924=DIRECTION('center_axis',(1.,0.,-2.89120579329468E-17));
#104925=DIRECTION('ref_axis',(-2.89120579329468E-17,0.,-1.));
#104926=DIRECTION('center_axis',(1.,0.,-5.33761069531325E-17));
#104927=DIRECTION('ref_axis',(-5.33761069531325E-17,0.,-1.));
#104928=DIRECTION('',(1.,0.,-2.89120579329468E-17));
#104929=DIRECTION('center_axis',(1.,0.,-2.89120579329468E-17));
#104930=DIRECTION('ref_axis',(-2.89120579329468E-17,0.,-1.));
#104931=DIRECTION('center_axis',(1.,0.,-2.89120579329468E-17));
#104932=DIRECTION('ref_axis',(-2.89120579329468E-17,0.,-1.));
#104933=DIRECTION('center_axis',(1.,0.,-5.33761069531325E-17));
#104934=DIRECTION('ref_axis',(-5.33761069531325E-17,0.,-1.));
#104935=DIRECTION('',(1.,0.,-2.89120579329468E-17));
#104936=DIRECTION('center_axis',(1.,0.,-2.89120579329468E-17));
#104937=DIRECTION('ref_axis',(-2.89120579329468E-17,0.,-1.));
#104938=DIRECTION('center_axis',(1.,0.,-2.89120579329468E-17));
#104939=DIRECTION('ref_axis',(-2.89120579329468E-17,0.,-1.));
#104940=DIRECTION('center_axis',(1.,0.,-5.33761069531325E-17));
#104941=DIRECTION('ref_axis',(-5.33761069531325E-17,0.,-1.));
#104942=DIRECTION('',(1.,0.,-2.89120579329468E-17));
#104943=DIRECTION('center_axis',(1.,0.,-2.89120579329468E-17));
#104944=DIRECTION('ref_axis',(-2.89120579329468E-17,0.,-1.));
#104945=DIRECTION('center_axis',(1.,0.,-2.89120579329468E-17));
#104946=DIRECTION('ref_axis',(-2.89120579329468E-17,0.,-1.));
#104947=DIRECTION('center_axis',(1.,0.,-5.33761069531325E-17));
#104948=DIRECTION('ref_axis',(-5.33761069531325E-17,0.,-1.));
#104949=DIRECTION('',(1.,0.,-2.89120579329468E-17));
#104950=DIRECTION('center_axis',(1.,0.,-2.89120579329468E-17));
#104951=DIRECTION('ref_axis',(-2.89120579329468E-17,0.,-1.));
#104952=DIRECTION('center_axis',(-1.,0.,0.));
#104953=DIRECTION('ref_axis',(0.,0.,1.));
#104954=DIRECTION('',(0.,0.,-1.));
#104955=DIRECTION('',(0.,-1.,0.));
#104956=DIRECTION('',(0.,0.,-1.));
#104957=DIRECTION('',(0.,-1.,0.));
#104958=DIRECTION('center_axis',(1.22464679914735E-16,0.,1.));
#104959=DIRECTION('ref_axis',(1.,0.,-1.22464679914735E-16));
#104960=DIRECTION('',(-1.,0.,1.22464679914735E-16));
#104961=DIRECTION('',(0.,1.,0.));
#104962=DIRECTION('',(-1.,0.,1.22464679914735E-16));
#104963=DIRECTION('center_axis',(1.,0.,-5.33761069531325E-17));
#104964=DIRECTION('ref_axis',(-5.33761069531325E-17,0.,-1.));
#104965=DIRECTION('',(5.33761069531325E-17,0.,1.));
#104966=DIRECTION('',(0.,1.,0.));
#104967=DIRECTION('',(5.33761069531325E-17,0.,1.));
#104968=DIRECTION('',(0.,-1.,0.));
#104969=DIRECTION('center_axis',(0.,0.,-1.));
#104970=DIRECTION('ref_axis',(-1.,0.,0.));
#104971=DIRECTION('',(1.,0.,0.));
#104972=DIRECTION('',(0.,-1.,0.));
#104973=DIRECTION('',(1.,0.,0.));
#104974=DIRECTION('',(0.,-1.,0.));
#104975=DIRECTION('center_axis',(-1.,0.,0.));
#104976=DIRECTION('ref_axis',(0.,0.,1.));
#104977=DIRECTION('',(0.,0.,-1.));
#104978=DIRECTION('',(0.,-1.,0.));
#104979=DIRECTION('',(0.,0.,-1.));
#104980=DIRECTION('center_axis',(0.,0.,1.));
#104981=DIRECTION('ref_axis',(1.,0.,0.));
#104982=DIRECTION('',(-1.,0.,0.));
#104983=DIRECTION('',(0.,1.,0.));
#104984=DIRECTION('',(-1.,0.,0.));
#104985=DIRECTION('center_axis',(-1.,0.,5.78241158658936E-17));
#104986=DIRECTION('ref_axis',(5.78241158658936E-17,0.,1.));
#104987=DIRECTION('',(-5.78241158658936E-17,0.,-1.));
#104988=DIRECTION('',(0.,1.,0.));
#104989=DIRECTION('',(-5.78241158658936E-17,0.,-1.));
#104990=DIRECTION('',(0.,-1.,0.));
#104991=DIRECTION('center_axis',(-7.70988211545248E-17,0.,-1.));
#104992=DIRECTION('ref_axis',(-1.,0.,7.70988211545248E-17));
#104993=DIRECTION('',(1.,0.,-7.70988211545248E-17));
#104994=DIRECTION('',(0.,-1.,0.));
#104995=DIRECTION('',(1.,0.,-7.70988211545248E-17));
#104996=DIRECTION('center_axis',(0.,1.,0.));
#104997=DIRECTION('ref_axis',(0.,0.,1.));
#104998=DIRECTION('center_axis',(0.,1.,0.));
#104999=DIRECTION('ref_axis',(0.,0.,1.));
#105000=DIRECTION('center_axis',(0.,-1.,0.));
#105001=DIRECTION('ref_axis',(0.,0.,1.));
#105002=DIRECTION('center_axis',(0.,-1.,0.));
#105003=DIRECTION('ref_axis',(0.,0.,1.));
#105004=DIRECTION('center_axis',(0.,1.,0.));
#105005=DIRECTION('ref_axis',(0.,0.,1.));
#105006=DIRECTION('center_axis',(0.,1.,0.));
#105007=DIRECTION('ref_axis',(0.,0.,1.));
#105008=DIRECTION('center_axis',(0.,-1.,0.));
#105009=DIRECTION('ref_axis',(0.,0.,1.));
#105010=DIRECTION('center_axis',(0.,-1.,0.));
#105011=DIRECTION('ref_axis',(0.,0.,1.));
#105012=DIRECTION('center_axis',(0.,1.,0.));
#105013=DIRECTION('ref_axis',(0.,0.,1.));
#105014=DIRECTION('center_axis',(0.,1.,0.));
#105015=DIRECTION('ref_axis',(0.,0.,1.));
#105016=DIRECTION('center_axis',(0.,-1.,0.));
#105017=DIRECTION('ref_axis',(0.,0.,-1.));
#105018=DIRECTION('center_axis',(0.,-1.,0.));
#105019=DIRECTION('ref_axis',(0.,0.,-1.));
#105020=DIRECTION('center_axis',(0.,1.,0.));
#105021=DIRECTION('ref_axis',(0.,0.,1.));
#105022=DIRECTION('center_axis',(0.,1.,0.));
#105023=DIRECTION('ref_axis',(0.,0.,1.));
#131014=CARTESIAN_POINT('',(0.,0.,0.));
#131015=CARTESIAN_POINT('Origin',(-55.,-786.679542586191,65.));
#131016=CARTESIAN_POINT('',(-50.,-786.679542586191,72.5));
#131017=CARTESIAN_POINT('Origin',(-50.,-786.679542586191,65.));
#131018=CARTESIAN_POINT('',(-45.,-786.679542586191,72.5));
#131019=CARTESIAN_POINT('',(-55.,-786.679542586191,72.5));
#131020=CARTESIAN_POINT('Origin',(-45.,-786.679542586191,65.));
#131021=CARTESIAN_POINT('Origin',(-55.,-646.67954258619,65.));
#131022=CARTESIAN_POINT('',(-50.,-646.67954258619,72.5));
#131023=CARTESIAN_POINT('Origin',(-50.,-646.67954258619,65.));
#131024=CARTESIAN_POINT('',(-45.,-646.67954258619,72.5));
#131025=CARTESIAN_POINT('',(-55.,-646.67954258619,72.5));
#131026=CARTESIAN_POINT('Origin',(-45.,-646.67954258619,65.));
#131027=CARTESIAN_POINT('Origin',(-55.,-506.67954258619,65.));
#131028=CARTESIAN_POINT('',(-50.,-506.67954258619,72.5));
#131029=CARTESIAN_POINT('Origin',(-50.,-506.67954258619,65.));
#131030=CARTESIAN_POINT('',(-45.,-506.67954258619,72.5));
#131031=CARTESIAN_POINT('',(-55.,-506.67954258619,72.5));
#131032=CARTESIAN_POINT('Origin',(-45.,-506.67954258619,65.));
#131033=CARTESIAN_POINT('Origin',(-55.,-366.67954258619,65.));
#131034=CARTESIAN_POINT('',(-50.,-366.67954258619,72.5));
#131035=CARTESIAN_POINT('Origin',(-50.,-366.67954258619,65.));
#131036=CARTESIAN_POINT('',(-45.,-366.67954258619,72.5));
#131037=CARTESIAN_POINT('',(-55.,-366.67954258619,72.5));
#131038=CARTESIAN_POINT('Origin',(-45.,-366.67954258619,65.));
#131039=CARTESIAN_POINT('Origin',(-55.,-226.67954258619,65.));
#131040=CARTESIAN_POINT('',(-50.,-226.67954258619,72.5));
#131041=CARTESIAN_POINT('Origin',(-50.,-226.67954258619,65.));
#131042=CARTESIAN_POINT('',(-45.,-226.67954258619,72.5));
#131043=CARTESIAN_POINT('',(-55.,-226.67954258619,72.5));
#131044=CARTESIAN_POINT('Origin',(-45.,-226.67954258619,65.));
#131045=CARTESIAN_POINT('Origin',(-55.,-86.6795425861914,65.));
#131046=CARTESIAN_POINT('',(-50.,-86.6795425861914,72.5));
#131047=CARTESIAN_POINT('Origin',(-50.,-86.6795425861914,65.));
#131048=CARTESIAN_POINT('',(-45.,-86.6795425861914,72.5));
#131049=CARTESIAN_POINT('',(-55.,-86.6795425861914,72.5));
#131050=CARTESIAN_POINT('Origin',(-45.,-86.6795425861914,65.));
#131051=CARTESIAN_POINT('Origin',(-55.,53.3204574138085,65.));
#131052=CARTESIAN_POINT('',(-50.,53.3204574138085,72.5));
#131053=CARTESIAN_POINT('Origin',(-50.,53.3204574138085,65.));
#131054=CARTESIAN_POINT('',(-45.,53.3204574138085,72.5));
#131055=CARTESIAN_POINT('',(-55.,53.3204574138085,72.5));
#131056=CARTESIAN_POINT('Origin',(-45.,53.3204574138085,65.));
#131057=CARTESIAN_POINT('Origin',(-55.,193.320457413809,65.));
#131058=CARTESIAN_POINT('',(-50.,193.320457413809,72.5));
#131059=CARTESIAN_POINT('Origin',(-50.,193.320457413809,65.));
#131060=CARTESIAN_POINT('',(-45.,193.320457413809,72.5));
#131061=CARTESIAN_POINT('',(-55.,193.320457413809,72.5));
#131062=CARTESIAN_POINT('Origin',(-45.,193.320457413809,65.));
#131063=CARTESIAN_POINT('Origin',(-55.,333.32045741381,65.));
#131064=CARTESIAN_POINT('',(-50.,333.32045741381,72.5));
#131065=CARTESIAN_POINT('Origin',(-50.,333.32045741381,65.));
#131066=CARTESIAN_POINT('',(-45.,333.32045741381,72.5));
#131067=CARTESIAN_POINT('',(-55.,333.32045741381,72.5));
#131068=CARTESIAN_POINT('Origin',(-45.,333.32045741381,65.));
#131069=CARTESIAN_POINT('Origin',(-55.,473.320457413809,65.));
#131070=CARTESIAN_POINT('',(-50.,473.320457413809,72.5));
#131071=CARTESIAN_POINT('Origin',(-50.,473.320457413809,65.));
#131072=CARTESIAN_POINT('',(-45.,473.320457413809,72.5));
#131073=CARTESIAN_POINT('',(-55.,473.320457413809,72.5));
#131074=CARTESIAN_POINT('Origin',(-45.,473.320457413809,65.));
#131075=CARTESIAN_POINT('Origin',(-55.,613.320457413809,65.));
#131076=CARTESIAN_POINT('',(-50.,613.320457413809,72.5));
#131077=CARTESIAN_POINT('Origin',(-50.,613.320457413809,65.));
#131078=CARTESIAN_POINT('',(-45.,613.320457413809,72.5));
#131079=CARTESIAN_POINT('',(-55.,613.320457413809,72.5));
#131080=CARTESIAN_POINT('Origin',(-45.,613.320457413809,65.));
#131081=CARTESIAN_POINT('Origin',(-55.,753.32045741381,65.));
#131082=CARTESIAN_POINT('',(-50.,753.32045741381,72.5));
#131083=CARTESIAN_POINT('Origin',(-50.,753.32045741381,65.));
#131084=CARTESIAN_POINT('',(-45.,753.32045741381,72.5));
#131085=CARTESIAN_POINT('',(-55.,753.32045741381,72.5));
#131086=CARTESIAN_POINT('Origin',(-45.,753.32045741381,65.));
#131087=CARTESIAN_POINT('Origin',(0.,900.,5.));
#131088=CARTESIAN_POINT('',(0.,-900.,5.));
#131089=CARTESIAN_POINT('',(0.,-900.,0.));
#131090=CARTESIAN_POINT('',(0.,-900.,5.));
#131091=CARTESIAN_POINT('',(0.,900.,0.));
#131092=CARTESIAN_POINT('',(0.,900.,0.));
#131093=CARTESIAN_POINT('',(0.,900.,5.));
#131094=CARTESIAN_POINT('',(0.,900.,5.));
#131095=CARTESIAN_POINT('',(0.,900.,5.));
#131096=CARTESIAN_POINT('Origin',(0.,900.,0.));
#131097=CARTESIAN_POINT('',(-48.,-900.,5.8783046359073E-15));
#131098=CARTESIAN_POINT('',(0.,-900.,0.));
#131099=CARTESIAN_POINT('',(-48.,900.,5.8783046359073E-15));
#131100=CARTESIAN_POINT('',(-48.,900.,5.8783046359073E-15));
#131101=CARTESIAN_POINT('',(0.,900.,0.));
#131102=CARTESIAN_POINT('Origin',(-50.,900.,6.12323399573677E-15));
#131103=CARTESIAN_POINT('',(-50.,-900.,2.00000000000001));
#131104=CARTESIAN_POINT('',(-50.,-900.,128.));
#131105=CARTESIAN_POINT('',(-50.,-900.,6.12323399573677E-15));
#131106=CARTESIAN_POINT('',(-50.,900.,128.));
#131107=CARTESIAN_POINT('',(-50.,900.,128.));
#131108=CARTESIAN_POINT('',(-50.,900.,2.00000000000001));
#131109=CARTESIAN_POINT('',(-50.,900.,6.12323399573677E-15));
#131110=CARTESIAN_POINT('',(-50.,900.,2.00000000000001));
#131111=CARTESIAN_POINT('Origin',(-50.,900.,130.));
#131112=CARTESIAN_POINT('',(-48.,900.,130.));
#131113=CARTESIAN_POINT('',(0.,900.,130.));
#131114=CARTESIAN_POINT('',(-50.,900.,130.));
#131115=CARTESIAN_POINT('',(-48.,-900.,130.));
#131116=CARTESIAN_POINT('',(-48.,900.,130.));
#131117=CARTESIAN_POINT('',(0.,-900.,130.));
#131118=CARTESIAN_POINT('',(-50.,-900.,130.));
#131119=CARTESIAN_POINT('',(0.,900.,130.));
#131120=CARTESIAN_POINT('Origin',(0.,900.,130.));
#131121=CARTESIAN_POINT('',(0.,-900.,125.));
#131122=CARTESIAN_POINT('',(0.,-900.,130.));
#131123=CARTESIAN_POINT('',(0.,900.,125.));
#131124=CARTESIAN_POINT('',(0.,900.,125.));
#131125=CARTESIAN_POINT('',(0.,900.,130.));
#131126=CARTESIAN_POINT('Origin',(0.,900.,125.));
#131127=CARTESIAN_POINT('',(-43.,-900.,125.));
#131128=CARTESIAN_POINT('',(0.,-900.,125.));
#131129=CARTESIAN_POINT('',(-43.,900.,125.));
#131130=CARTESIAN_POINT('',(-43.,900.,125.));
#131131=CARTESIAN_POINT('',(0.,900.,125.));
#131132=CARTESIAN_POINT('Origin',(-45.,900.,125.));
#131133=CARTESIAN_POINT('',(-45.,-900.,123.));
#131134=CARTESIAN_POINT('',(-45.,-900.,7.00000000000001));
#131135=CARTESIAN_POINT('',(-45.,-900.,125.));
#131136=CARTESIAN_POINT('',(-45.,900.,7.00000000000001));
#131137=CARTESIAN_POINT('',(-45.,900.,7.));
#131138=CARTESIAN_POINT('',(-45.,900.,123.));
#131139=CARTESIAN_POINT('',(-45.,900.,125.));
#131140=CARTESIAN_POINT('',(-45.,-900.,123.));
#131141=CARTESIAN_POINT('Origin',(-45.,900.,5.));
#131142=CARTESIAN_POINT('',(-43.,900.,5.));
#131143=CARTESIAN_POINT('',(-45.,900.,5.));
#131144=CARTESIAN_POINT('',(-43.,-900.,5.));
#131145=CARTESIAN_POINT('',(-43.,-900.,5.));
#131146=CARTESIAN_POINT('',(-45.,-900.,5.));
#131147=CARTESIAN_POINT('Origin',(0.,900.,0.));
#131148=CARTESIAN_POINT('Origin',(-48.,900.,128.));
#131149=CARTESIAN_POINT('Origin',(-43.,900.,123.));
#131150=CARTESIAN_POINT('Origin',(-43.,900.,7.));
#131151=CARTESIAN_POINT('Origin',(-48.,900.,2.00000000000001));
#131152=CARTESIAN_POINT('Origin',(0.,-900.,0.));
#131153=CARTESIAN_POINT('Origin',(-48.,-900.,128.));
#131154=CARTESIAN_POINT('Origin',(-48.,-900.,2.00000000000001));
#131155=CARTESIAN_POINT('Origin',(-43.,-900.,7.));
#131156=CARTESIAN_POINT('Origin',(-43.,-900.,123.));
#131157=CARTESIAN_POINT('Origin',(-48.,900.,128.));
#131158=CARTESIAN_POINT('Origin',(-48.,900.,2.00000000000001));
#131159=CARTESIAN_POINT('Origin',(-43.,900.,7.));
#131160=CARTESIAN_POINT('Origin',(-43.,900.,123.));
#310581=UNCERTAINTY_MEASURE_WITH_UNIT(LENGTH_MEASURE(0.01),#310624,
'DISTANCE_ACCURACY_VALUE',
'Maximum model space distance between geometric entities at asserted c
onnectivities');
#310601=UNCERTAINTY_MEASURE_WITH_UNIT(LENGTH_MEASURE(0.01),#310624,
'DISTANCE_ACCURACY_VALUE',
'Maximum model space distance between geometric entities at asserted c
onnectivities');
#310603=(
GEOMETRIC_REPRESENTATION_CONTEXT(3)
GLOBAL_UNCERTAINTY_ASSIGNED_CONTEXT((#310581))
GLOBAL_UNIT_ASSIGNED_CONTEXT((#310624,#310626,#310627))
REPRESENTATION_CONTEXT('','3D')
);
#310623=(
GEOMETRIC_REPRESENTATION_CONTEXT(3)
GLOBAL_UNCERTAINTY_ASSIGNED_CONTEXT((#310601))
GLOBAL_UNIT_ASSIGNED_CONTEXT((#310624,#310626,#310627))
REPRESENTATION_CONTEXT('','3D')
);
#310624=(
LENGTH_UNIT()
NAMED_UNIT(*)
SI_UNIT(.MILLI.,.METRE.)
);
#310626=(
NAMED_UNIT(*)
PLANE_ANGLE_UNIT()
SI_UNIT($,.RADIAN.)
);
#310627=(
NAMED_UNIT(*)
SI_UNIT($,.STERADIAN.)
SOLID_ANGLE_UNIT()
);
#310629=SHAPE_DEFINITION_REPRESENTATION(#310650,#310894);
#310650=PRODUCT_DEFINITION_SHAPE('',$,#310916);
#310894=SHAPE_REPRESENTATION('',(#93964),#310603);
#310914=PRODUCT_DEFINITION_CONTEXT('part definition',#310979,'design');
#310916=PRODUCT_DEFINITION('Right Side Channel Support Rail',
'Right Side Channel Support Rail',#310937,#310914);
#310937=PRODUCT_DEFINITION_FORMATION('',$,#310982);
#310979=APPLICATION_CONTEXT(
'Core Data for Automotive Mechanical Design Process');
#310980=PRODUCT_CONTEXT('part definition',#310979,'mechanical');
#310982=PRODUCT('Right Side Channel Support Rail',
'Right Side Channel Support Rail',$,(#310980));
#311003=PRESENTATION_STYLE_ASSIGNMENT((#311010));
#311010=SURFACE_STYLE_USAGE(.BOTH.,#311017);
#311017=SURFACE_SIDE_STYLE('',(#311024));
#311024=SURFACE_STYLE_FILL_AREA(#311031);
#311031=FILL_AREA_STYLE('Opaque(97,158,199)',(#311038));
#311038=FILL_AREA_STYLE_COLOUR('Opaque(97,158,199)',#311045);
#311045=COLOUR_RGB('Opaque(97,158,199)',0.380392156862745,0.619607843137255,
0.780392156862745);
ENDSEC;
END-ISO-10303-21;
